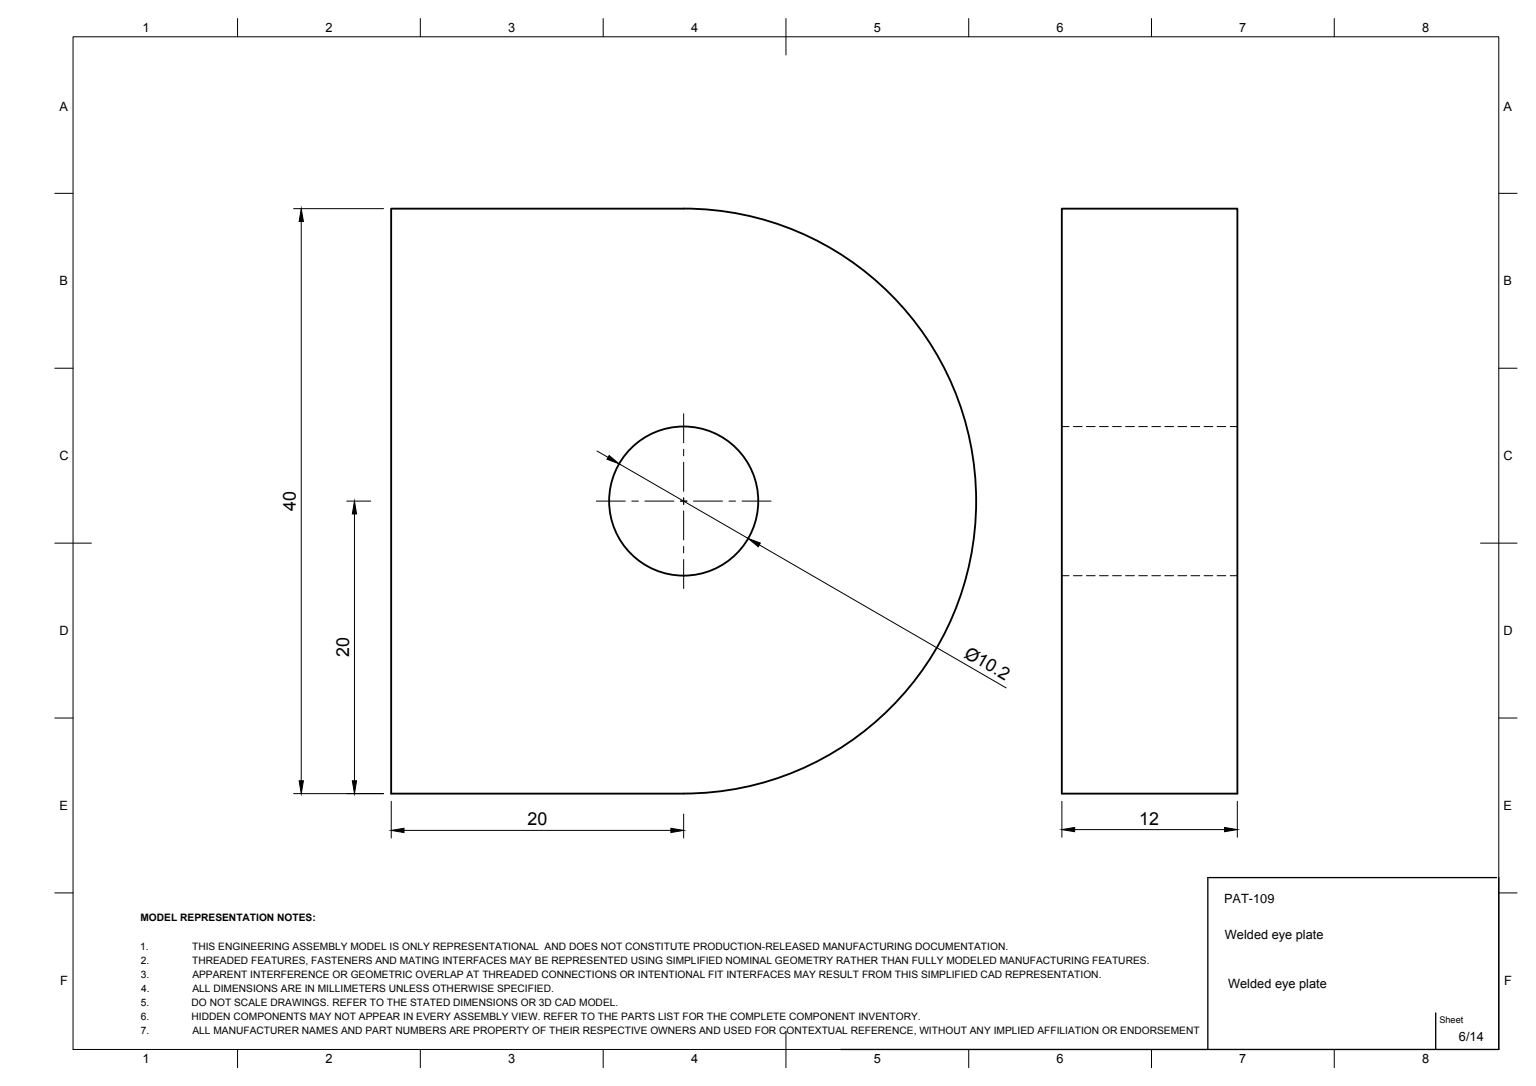
ISO-10303-21;
HEADER;
/* Generated by software containing ST-Developer
 * from STEP Tools, Inc. (www.steptools.com) 
 */

FILE_DESCRIPTION(
/* description */ ('Twin-shackle spreader bar'),
/* implementation_level */ '2;1');

FILE_NAME(
/* name */ 'Welded eye plate.step',
/* time_stamp */ '2026-10-27T20:18:10-07:00',
/* author */ (''),
/* organization */ (''),
/* preprocessor_version */ 'ST-DEVELOPER v20.2',
/* originating_system */ 'Autodesk Translation Framework v15.17.0.0',
/* authorisation */ '');

FILE_SCHEMA (('AUTOMOTIVE_DESIGN { 1 0 10303 214 3 1 1 }'));
ENDSEC;

DATA;
#10=MECHANICAL_DESIGN_GEOMETRIC_PRESENTATION_REPRESENTATION('',(#158),#1829);
#104=CIRCLE('',#1037,0.510000000000002);
#105=CIRCLE('',#1038,0.510000000000002);
#106=CIRCLE('',#1043,2.);
#107=CIRCLE('',#1045,2.);
#131=CYLINDRICAL_SURFACE('',#1036,0.510000000000002);
#132=CYLINDRICAL_SURFACE('',#1044,2.);
#144=SHAPE_REPRESENTATION_RELATIONSHIP('SRR','None',#1880,#151);
#151=ADVANCED_BREP_SHAPE_REPRESENTATION('',(#165),#1821);
#158=STYLED_ITEM('',(#1977),#165);
#165=MANIFOLD_SOLID_BREP('Body1',#938);
#173=FACE_BOUND('',#253,.T.);
#174=FACE_BOUND('',#256,.T.);
#196=FACE_OUTER_BOUND('',#248,.T.);
#197=FACE_OUTER_BOUND('',#249,.T.);
#198=FACE_OUTER_BOUND('',#250,.T.);
#199=FACE_OUTER_BOUND('',#251,.T.);
#200=FACE_OUTER_BOUND('',#252,.T.);
#201=FACE_OUTER_BOUND('',#254,.T.);
#202=FACE_OUTER_BOUND('',#255,.T.);
#248=EDGE_LOOP('',(#682,#683,#684,#685));
#249=EDGE_LOOP('',(#686,#687,#688,#689));
#250=EDGE_LOOP('',(#690,#691,#692,#693));
#251=EDGE_LOOP('',(#694,#695,#696,#697));
#252=EDGE_LOOP('',(#698,#699,#700,#701));
#253=EDGE_LOOP('',(#702));
#254=EDGE_LOOP('',(#703,#704,#705,#706));
#255=EDGE_LOOP('',(#707,#708,#709,#710));
#256=EDGE_LOOP('',(#711));
#325=LINE('',#1483,#401);
#326=LINE('',#1488,#402);
#327=LINE('',#1490,#403);
#328=LINE('',#1492,#404);
#329=LINE('',#1493,#405);
#330=LINE('',#1497,#406);
#331=LINE('',#1499,#407);
#332=LINE('',#1501,#408);
#333=LINE('',#1502,#409);
#334=LINE('',#1504,#410);
#335=LINE('',#1505,#411);
#401=VECTOR('',#1187,0.510000000000002);
#402=VECTOR('',#1192,1.);
#403=VECTOR('',#1193,1.);
#404=VECTOR('',#1194,1.);
#405=VECTOR('',#1195,1.);
#406=VECTOR('',#1198,1.);
#407=VECTOR('',#1199,1.);
#408=VECTOR('',#1200,1.);
#409=VECTOR('',#1201,1.);
#410=VECTOR('',#1204,1.);
#411=VECTOR('',#1205,1.);
#469=VERTEX_POINT('',#1480);
#470=VERTEX_POINT('',#1482);
#471=VERTEX_POINT('',#1486);
#472=VERTEX_POINT('',#1487);
#473=VERTEX_POINT('',#1489);
#474=VERTEX_POINT('',#1491);
#475=VERTEX_POINT('',#1495);
#476=VERTEX_POINT('',#1496);
#477=VERTEX_POINT('',#1498);
#478=VERTEX_POINT('',#1500);
#549=EDGE_CURVE('',#469,#469,#104,.T.);
#550=EDGE_CURVE('',#469,#470,#325,.T.);
#551=EDGE_CURVE('',#470,#470,#105,.T.);
#552=EDGE_CURVE('',#471,#472,#326,.T.);
#553=EDGE_CURVE('',#471,#473,#327,.T.);
#554=EDGE_CURVE('',#474,#473,#328,.T.);
#555=EDGE_CURVE('',#472,#474,#329,.T.);
#556=EDGE_CURVE('',#475,#476,#330,.T.);
#557=EDGE_CURVE('',#477,#475,#331,.T.);
#558=EDGE_CURVE('',#478,#477,#332,.T.);
#559=EDGE_CURVE('',#476,#478,#333,.T.);
#560=EDGE_CURVE('',#473,#478,#334,.T.);
#561=EDGE_CURVE('',#476,#471,#335,.T.);
#562=EDGE_CURVE('',#477,#474,#106,.T.);
#563=EDGE_CURVE('',#475,#472,#107,.T.);
#682=ORIENTED_EDGE('',*,*,#549,.F.);
#683=ORIENTED_EDGE('',*,*,#550,.T.);
#684=ORIENTED_EDGE('',*,*,#551,.F.);
#685=ORIENTED_EDGE('',*,*,#550,.F.);
#686=ORIENTED_EDGE('',*,*,#552,.F.);
#687=ORIENTED_EDGE('',*,*,#553,.T.);
#688=ORIENTED_EDGE('',*,*,#554,.F.);
#689=ORIENTED_EDGE('',*,*,#555,.F.);
#690=ORIENTED_EDGE('',*,*,#556,.F.);
#691=ORIENTED_EDGE('',*,*,#557,.F.);
#692=ORIENTED_EDGE('',*,*,#558,.F.);
#693=ORIENTED_EDGE('',*,*,#559,.F.);
#694=ORIENTED_EDGE('',*,*,#560,.F.);
#695=ORIENTED_EDGE('',*,*,#553,.F.);
#696=ORIENTED_EDGE('',*,*,#561,.F.);
#697=ORIENTED_EDGE('',*,*,#559,.T.);
#698=ORIENTED_EDGE('',*,*,#562,.T.);
#699=ORIENTED_EDGE('',*,*,#554,.T.);
#700=ORIENTED_EDGE('',*,*,#560,.T.);
#701=ORIENTED_EDGE('',*,*,#558,.T.);
#702=ORIENTED_EDGE('',*,*,#551,.T.);
#703=ORIENTED_EDGE('',*,*,#555,.T.);
#704=ORIENTED_EDGE('',*,*,#562,.F.);
#705=ORIENTED_EDGE('',*,*,#557,.T.);
#706=ORIENTED_EDGE('',*,*,#563,.T.);
#707=ORIENTED_EDGE('',*,*,#563,.F.);
#708=ORIENTED_EDGE('',*,*,#556,.T.);
#709=ORIENTED_EDGE('',*,*,#561,.T.);
#710=ORIENTED_EDGE('',*,*,#552,.T.);
#711=ORIENTED_EDGE('',*,*,#549,.T.);
#862=PLANE('',#1039);
#863=PLANE('',#1040);
#864=PLANE('',#1041);
#865=PLANE('',#1042);
#866=PLANE('',#1046);
#897=ADVANCED_FACE('',(#196),#131,.F.);
#898=ADVANCED_FACE('',(#197),#862,.T.);
#899=ADVANCED_FACE('',(#198),#863,.T.);
#900=ADVANCED_FACE('',(#199),#864,.T.);
#901=ADVANCED_FACE('',(#200,#173),#865,.T.);
#902=ADVANCED_FACE('',(#201),#132,.T.);
#903=ADVANCED_FACE('',(#202,#174),#866,.F.);
#938=CLOSED_SHELL('',(#897,#898,#899,#900,#901,#902,#903));
#1035=AXIS2_PLACEMENT_3D('',#1478,#1181,#1182);
#1036=AXIS2_PLACEMENT_3D('',#1479,#1183,#1184);
#1037=AXIS2_PLACEMENT_3D('',#1481,#1185,#1186);
#1038=AXIS2_PLACEMENT_3D('',#1484,#1188,#1189);
#1039=AXIS2_PLACEMENT_3D('',#1485,#1190,#1191);
#1040=AXIS2_PLACEMENT_3D('',#1494,#1196,#1197);
#1041=AXIS2_PLACEMENT_3D('',#1503,#1202,#1203);
#1042=AXIS2_PLACEMENT_3D('',#1506,#1206,#1207);
#1043=AXIS2_PLACEMENT_3D('',#1507,#1208,#1209);
#1044=AXIS2_PLACEMENT_3D('',#1508,#1210,#1211);
#1045=AXIS2_PLACEMENT_3D('',#1509,#1212,#1213);
#1046=AXIS2_PLACEMENT_3D('',#1510,#1214,#1215);
#1181=DIRECTION('axis',(0.,0.,1.));
#1182=DIRECTION('refdir',(1.,0.,0.));
#1183=DIRECTION('center_axis',(0.,1.,0.));
#1184=DIRECTION('ref_axis',(1.,0.,0.));
#1185=DIRECTION('center_axis',(0.,1.,0.));
#1186=DIRECTION('ref_axis',(1.,0.,0.));
#1187=DIRECTION('',(0.,1.,0.));
#1188=DIRECTION('center_axis',(0.,-1.,0.));
#1189=DIRECTION('ref_axis',(1.,0.,0.));
#1190=DIRECTION('center_axis',(-1.,0.,0.));
#1191=DIRECTION('ref_axis',(0.,0.,1.));
#1192=DIRECTION('',(0.,0.,-1.));
#1193=DIRECTION('',(0.,1.,0.));
#1194=DIRECTION('',(0.,0.,1.));
#1195=DIRECTION('',(0.,1.,0.));
#1196=DIRECTION('center_axis',(1.,0.,0.));
#1197=DIRECTION('ref_axis',(0.,0.,-1.));
#1198=DIRECTION('',(0.,0.,1.));
#1199=DIRECTION('',(0.,-1.,0.));
#1200=DIRECTION('',(0.,0.,-1.));
#1201=DIRECTION('',(0.,1.,0.));
#1202=DIRECTION('center_axis',(0.,0.,1.));
#1203=DIRECTION('ref_axis',(1.,0.,0.));
#1204=DIRECTION('',(1.,0.,0.));
#1205=DIRECTION('',(-1.,0.,0.));
#1206=DIRECTION('center_axis',(0.,1.,0.));
#1207=DIRECTION('ref_axis',(1.,0.,0.));
#1208=DIRECTION('center_axis',(0.,1.,0.));
#1209=DIRECTION('ref_axis',(1.,0.,0.));
#1210=DIRECTION('center_axis',(0.,1.,0.));
#1211=DIRECTION('ref_axis',(1.,0.,0.));
#1212=DIRECTION('center_axis',(0.,1.,0.));
#1213=DIRECTION('ref_axis',(1.,0.,0.));
#1214=DIRECTION('center_axis',(0.,1.,0.));
#1215=DIRECTION('ref_axis',(1.,0.,0.));
#1478=CARTESIAN_POINT('',(0.,0.,0.));
#1479=CARTESIAN_POINT('Origin',(-21.,-0.7,-2.));
#1480=CARTESIAN_POINT('',(-21.51,-0.6,-2.));
#1481=CARTESIAN_POINT('Origin',(-21.,-0.6,-2.));
#1482=CARTESIAN_POINT('',(-21.51,0.6,-2.));
#1483=CARTESIAN_POINT('',(-21.51,-0.7,-2.));
#1484=CARTESIAN_POINT('Origin',(-21.,0.6,-2.));
#1485=CARTESIAN_POINT('Origin',(-23.,-0.6,-2.));
#1486=CARTESIAN_POINT('',(-23.,-0.6,0.));
#1487=CARTESIAN_POINT('',(-23.,-0.6,-2.));
#1488=CARTESIAN_POINT('',(-23.,-0.6,0.));
#1489=CARTESIAN_POINT('',(-23.,0.6,0.));
#1490=CARTESIAN_POINT('',(-23.,-0.6,0.));
#1491=CARTESIAN_POINT('',(-23.,0.6,-2.));
#1492=CARTESIAN_POINT('',(-23.,0.6,0.));
#1493=CARTESIAN_POINT('',(-23.,-0.6,-2.));
#1494=CARTESIAN_POINT('Origin',(-19.,-0.6,0.));
#1495=CARTESIAN_POINT('',(-19.,-0.6,-2.));
#1496=CARTESIAN_POINT('',(-19.,-0.6,0.));
#1497=CARTESIAN_POINT('',(-19.,-0.6,-2.));
#1498=CARTESIAN_POINT('',(-19.,0.6,-2.));
#1499=CARTESIAN_POINT('',(-19.,-0.6,-2.));
#1500=CARTESIAN_POINT('',(-19.,0.6,0.));
#1501=CARTESIAN_POINT('',(-19.,0.6,-2.));
#1502=CARTESIAN_POINT('',(-19.,-0.6,0.));
#1503=CARTESIAN_POINT('Origin',(-23.,-0.6,0.));
#1504=CARTESIAN_POINT('',(-19.,0.6,0.));
#1505=CARTESIAN_POINT('',(-19.,-0.6,0.));
#1506=CARTESIAN_POINT('Origin',(-21.,0.6,-2.));
#1507=CARTESIAN_POINT('Origin',(-21.,0.6,-2.));
#1508=CARTESIAN_POINT('Origin',(-21.,-0.6,-2.));
#1509=CARTESIAN_POINT('Origin',(-21.,-0.6,-2.));
#1510=CARTESIAN_POINT('Origin',(-21.,-0.6,-2.));
#1809=UNCERTAINTY_MEASURE_WITH_UNIT(LENGTH_MEASURE(0.001),#1830,
'DISTANCE_ACCURACY_VALUE',
'Maximum model space distance between geometric entities at asserted c
onnectivities');
#1817=UNCERTAINTY_MEASURE_WITH_UNIT(LENGTH_MEASURE(0.001),#1830,
'DISTANCE_ACCURACY_VALUE',
'Maximum model space distance between geometric entities at asserted c
onnectivities');
#1821=(
GEOMETRIC_REPRESENTATION_CONTEXT(3)
GLOBAL_UNCERTAINTY_ASSIGNED_CONTEXT((#1809))
GLOBAL_UNIT_ASSIGNED_CONTEXT((#1830,#1832,#1833))
REPRESENTATION_CONTEXT('','3D')
);
#1829=(
GEOMETRIC_REPRESENTATION_CONTEXT(3)
GLOBAL_UNCERTAINTY_ASSIGNED_CONTEXT((#1817))
GLOBAL_UNIT_ASSIGNED_CONTEXT((#1830,#1832,#1833))
REPRESENTATION_CONTEXT('','3D')
);
#1830=(
LENGTH_UNIT()
NAMED_UNIT(*)
SI_UNIT(.CENTI.,.METRE.)
);
#1832=(
NAMED_UNIT(*)
PLANE_ANGLE_UNIT()
SI_UNIT($,.RADIAN.)
);
#1833=(
NAMED_UNIT(*)
SI_UNIT($,.STERADIAN.)
SOLID_ANGLE_UNIT()
);
#1837=SHAPE_DEFINITION_REPRESENTATION(#1848,#1880);
#1848=PRODUCT_DEFINITION_SHAPE('',$,#1892);
#1880=SHAPE_REPRESENTATION('',(#1035),#1821);
#1888=PRODUCT_DEFINITION_CONTEXT('part definition',#1923,'design');
#1892=PRODUCT_DEFINITION('Welded eye plate','Welded eye plate',#1903,#1888);
#1903=PRODUCT_DEFINITION_FORMATION('',$,#1928);
#1923=APPLICATION_CONTEXT(
'Core Data for Automotive Mechanical Design Process');
#1924=PRODUCT_CONTEXT('part definition',#1923,'mechanical');
#1928=PRODUCT('Welded eye plate','Welded eye plate','Welded eye plate',
(#1924));
#1971=COLOUR_RGB('Sky Blue',0.24,0.69,0.87);
#1972=FILL_AREA_STYLE_COLOUR('',#1971);
#1973=FILL_AREA_STYLE('',(#1972));
#1974=SURFACE_STYLE_FILL_AREA(#1973);
#1975=SURFACE_SIDE_STYLE('',(#1974));
#1976=SURFACE_STYLE_USAGE(.BOTH.,#1975);
#1977=PRESENTATION_STYLE_ASSIGNMENT((#1976));
ENDSEC;
END-ISO-10303-21;
